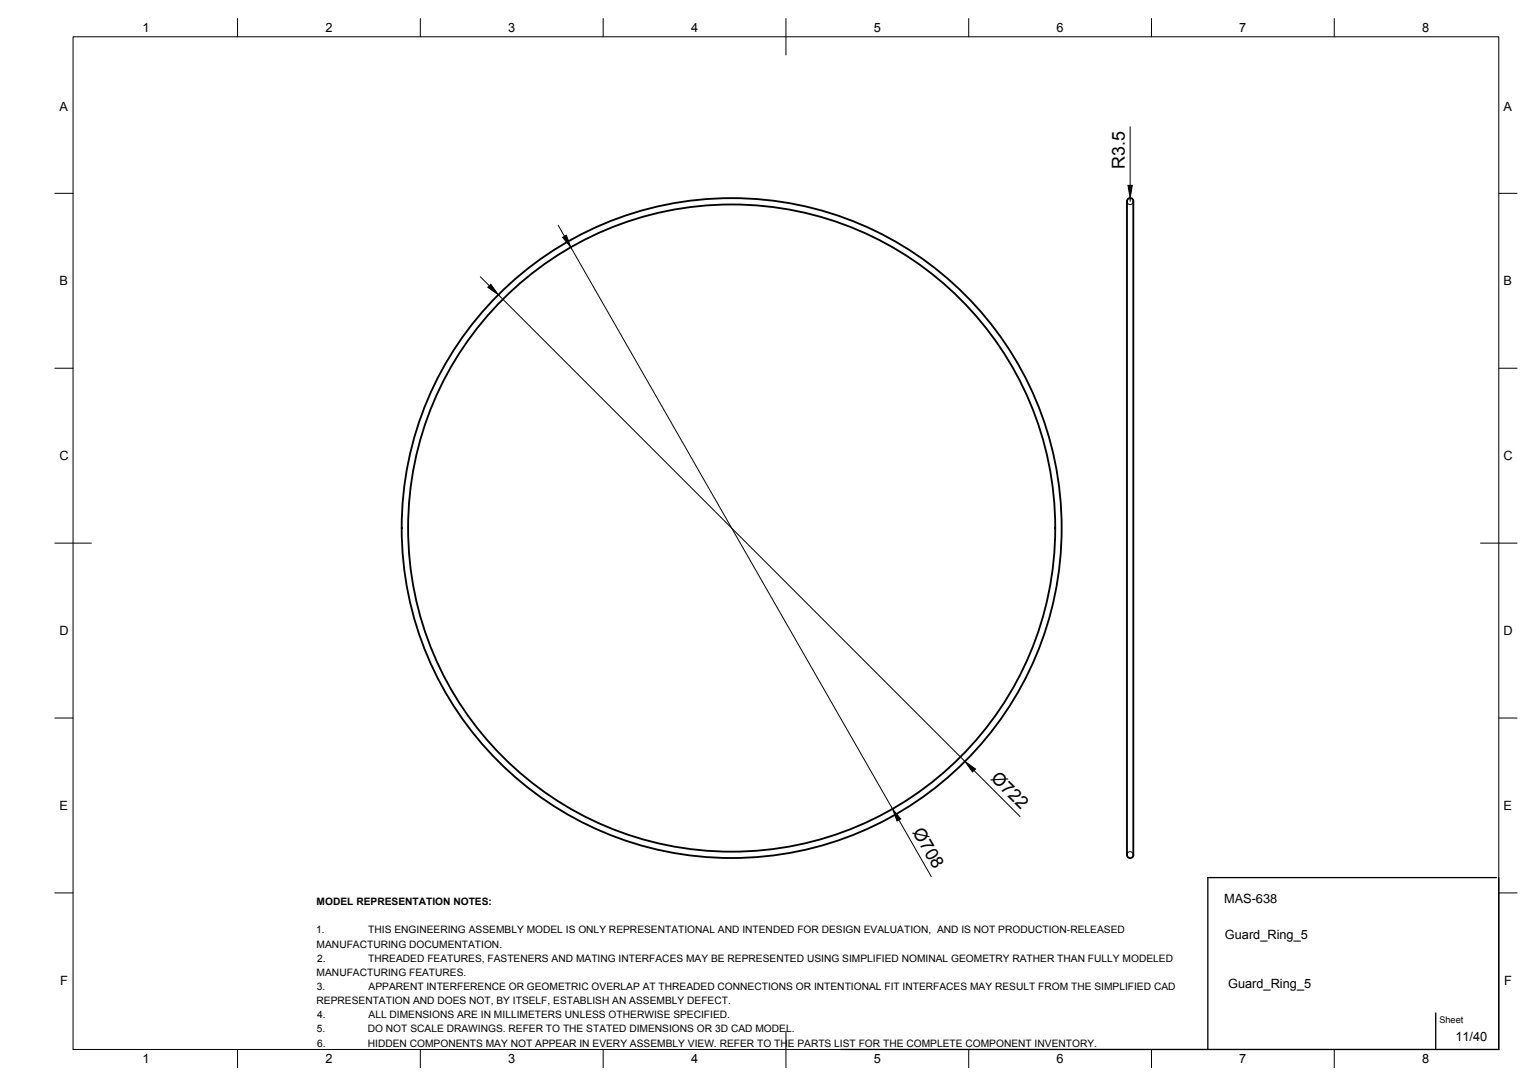
ISO-10303-21;
HEADER;
FILE_DESCRIPTION((''),'2;1');
FILE_NAME('Guard_Ring_5.step','2026-10-09T12:00:21-07:00',(''),(''),'','','');
FILE_SCHEMA (('AUTOMOTIVE_DESIGN { 1 0 10303 214 3 1 1 }'));
ENDSEC;
DATA;
#10=MECHANICAL_DESIGN_GEOMETRIC_PRESENTATION_REPRESENTATION('',(#402),#10334);
#338=SHAPE_REPRESENTATION_RELATIONSHIP('SRR','None',#10454,#370) ;
#370=ADVANCED_BREP_SHAPE_REPRESENTATION('',(#442),#10306) ;
#402=STYLED_ITEM('',(#10631),#442) ;
#442=MANIFOLD_SOLID_BREP('Body1',#3564) ;
#863=FACE_OUTER_BOUND('',#1063,.T.) ;
#1063=EDGE_LOOP('',(#2365,#2366,#2367,#2368)) ;
#1284=CIRCLE('',#3991,0.349999999999999) ;
#1285=CIRCLE('',#3992,35.4) ;
#1517=VERTEX_POINT('',#5673) ;
#1839=EDGE_CURVE('',#1517,#1517,#1284,.T.) ;
#1840=EDGE_CURVE('',#1517,#1517,#1285,.T.) ;
#2365=ORIENTED_EDGE('',*,*,#1839,.F.) ;
#2366=ORIENTED_EDGE('',*,*,#1840,.T.) ;
#2367=ORIENTED_EDGE('',*,*,#1839,.T.) ;
#2368=ORIENTED_EDGE('',*,*,#1840,.F.) ;
#3309=TOROIDAL_SURFACE('',#3990,35.75,0.349999999999999) ;
#3371=ADVANCED_FACE('',(#863),#3309,.T.) ;
#3564=CLOSED_SHELL('',(#3371)) ;
#3989=AXIS2_PLACEMENT_3D('',#5671,#4539,#4540) ;
#3990=AXIS2_PLACEMENT_3D('',#5672,#4541,#4542) ;
#3991=AXIS2_PLACEMENT_3D('',#5674,#4543,#4544) ;
#3992=AXIS2_PLACEMENT_3D('',#5675,#4545,#4546) ;
#4539=DIRECTION('axis',(0.,0.,1.)) ;
#4540=DIRECTION('refdir',(1.,0.,0.)) ;
#4541=DIRECTION('center_axis',(6.42891162084177E-17,1.,1.01883556321148E-16)) ;
#4542=DIRECTION('ref_axis',(-1.,0.,0.)) ;
#4543=DIRECTION('center_axis',(0.,1.01883556321148E-16,-1.)) ;
#4544=DIRECTION('ref_axis',(1.,0.,0.)) ;
#4545=DIRECTION('center_axis',(-6.42891162084177E-17,-1.,-1.01883556321148E-16)) ;
#4546=DIRECTION('ref_axis',(-1.,6.42891162084177E-17,6.55000379205715E-33)) ;
#5671=CARTESIAN_POINT('',(0.,0.,0.)) ;
#5672=CARTESIAN_POINT('Origin',(23.47768801576,65.9830586252741,68.2224337400009)) ;
#5673=CARTESIAN_POINT('',(58.87768801576,65.9830586252741,68.2224337400009)) ;
#5674=CARTESIAN_POINT('Origin',(59.22768801576,65.9830586252741,68.2224337400009)) ;
#5675=CARTESIAN_POINT('Origin',(23.47768801576,65.9830586252741,68.2224337400009)) ;
#10269=UNCERTAINTY_MEASURE_WITH_UNIT(LENGTH_MEASURE(0.001),#10335,
'DISTANCE_ACCURACY_VALUE',
'Maximum model space distance between geometric entities at asserted c
onnectivities') ;
#10297=UNCERTAINTY_MEASURE_WITH_UNIT(LENGTH_MEASURE(0.001),#10335,
'DISTANCE_ACCURACY_VALUE',
'Maximum model space distance between geometric entities at asserted c
onnectivities') ;
#10306=(
GEOMETRIC_REPRESENTATION_CONTEXT(3)
GLOBAL_UNCERTAINTY_ASSIGNED_CONTEXT((#10269))
GLOBAL_UNIT_ASSIGNED_CONTEXT((#10335,#10337,#10338))
REPRESENTATION_CONTEXT('','3D')
) ;
#10334=(
GEOMETRIC_REPRESENTATION_CONTEXT(3)
GLOBAL_UNCERTAINTY_ASSIGNED_CONTEXT((#10297))
GLOBAL_UNIT_ASSIGNED_CONTEXT((#10335,#10337,#10338))
REPRESENTATION_CONTEXT('','3D')
) ;
#10335=(
LENGTH_UNIT()
NAMED_UNIT(*)
SI_UNIT(.CENTI.,.METRE.)
) ;
#10337=(
NAMED_UNIT(*)
PLANE_ANGLE_UNIT()
SI_UNIT($,.RADIAN.)
) ;
#10338=(
NAMED_UNIT(*)
SI_UNIT($,.STERADIAN.)
SOLID_ANGLE_UNIT()
) ;
#10347=SHAPE_DEFINITION_REPRESENTATION(#10383,#10454) ;
#10383=PRODUCT_DEFINITION_SHAPE('',$,#10491) ;
#10454=SHAPE_REPRESENTATION('',(#3989),#10306) ;
#10482=PRODUCT_DEFINITION_CONTEXT('part definition',#10592,'design') ;
#10491=PRODUCT_DEFINITION('Guard_Ring_5','Guard_Ring_5',#10527,#10482) ;
#10527=PRODUCT_DEFINITION_FORMATION('',$,#10602) ;
#10592=APPLICATION_CONTEXT(
'Core Data for Automotive Mechanical Design Process') ;
#10593=PRODUCT_CONTEXT('part definition',#10592,'mechanical') ;
#10602=PRODUCT('Guard_Ring_5','Guard_Ring_5',$,(#10593)) ;
#10631=PRESENTATION_STYLE_ASSIGNMENT((#10635)) ;
#10635=SURFACE_STYLE_USAGE(.BOTH.,#10639) ;
#10639=SURFACE_SIDE_STYLE('',(#10643)) ;
#10643=SURFACE_STYLE_FILL_AREA(#10647) ;
#10647=FILL_AREA_STYLE('Opaque(25,25,25)',(#10651)) ;
#10651=FILL_AREA_STYLE_COLOUR('Opaque(25,25,25)',#10655) ;
#10655=COLOUR_RGB('Opaque(25,25,25)', 0.09019608, 0.27058824, 0.51372549) ;
ENDSEC;
END-ISO-10303-21;
